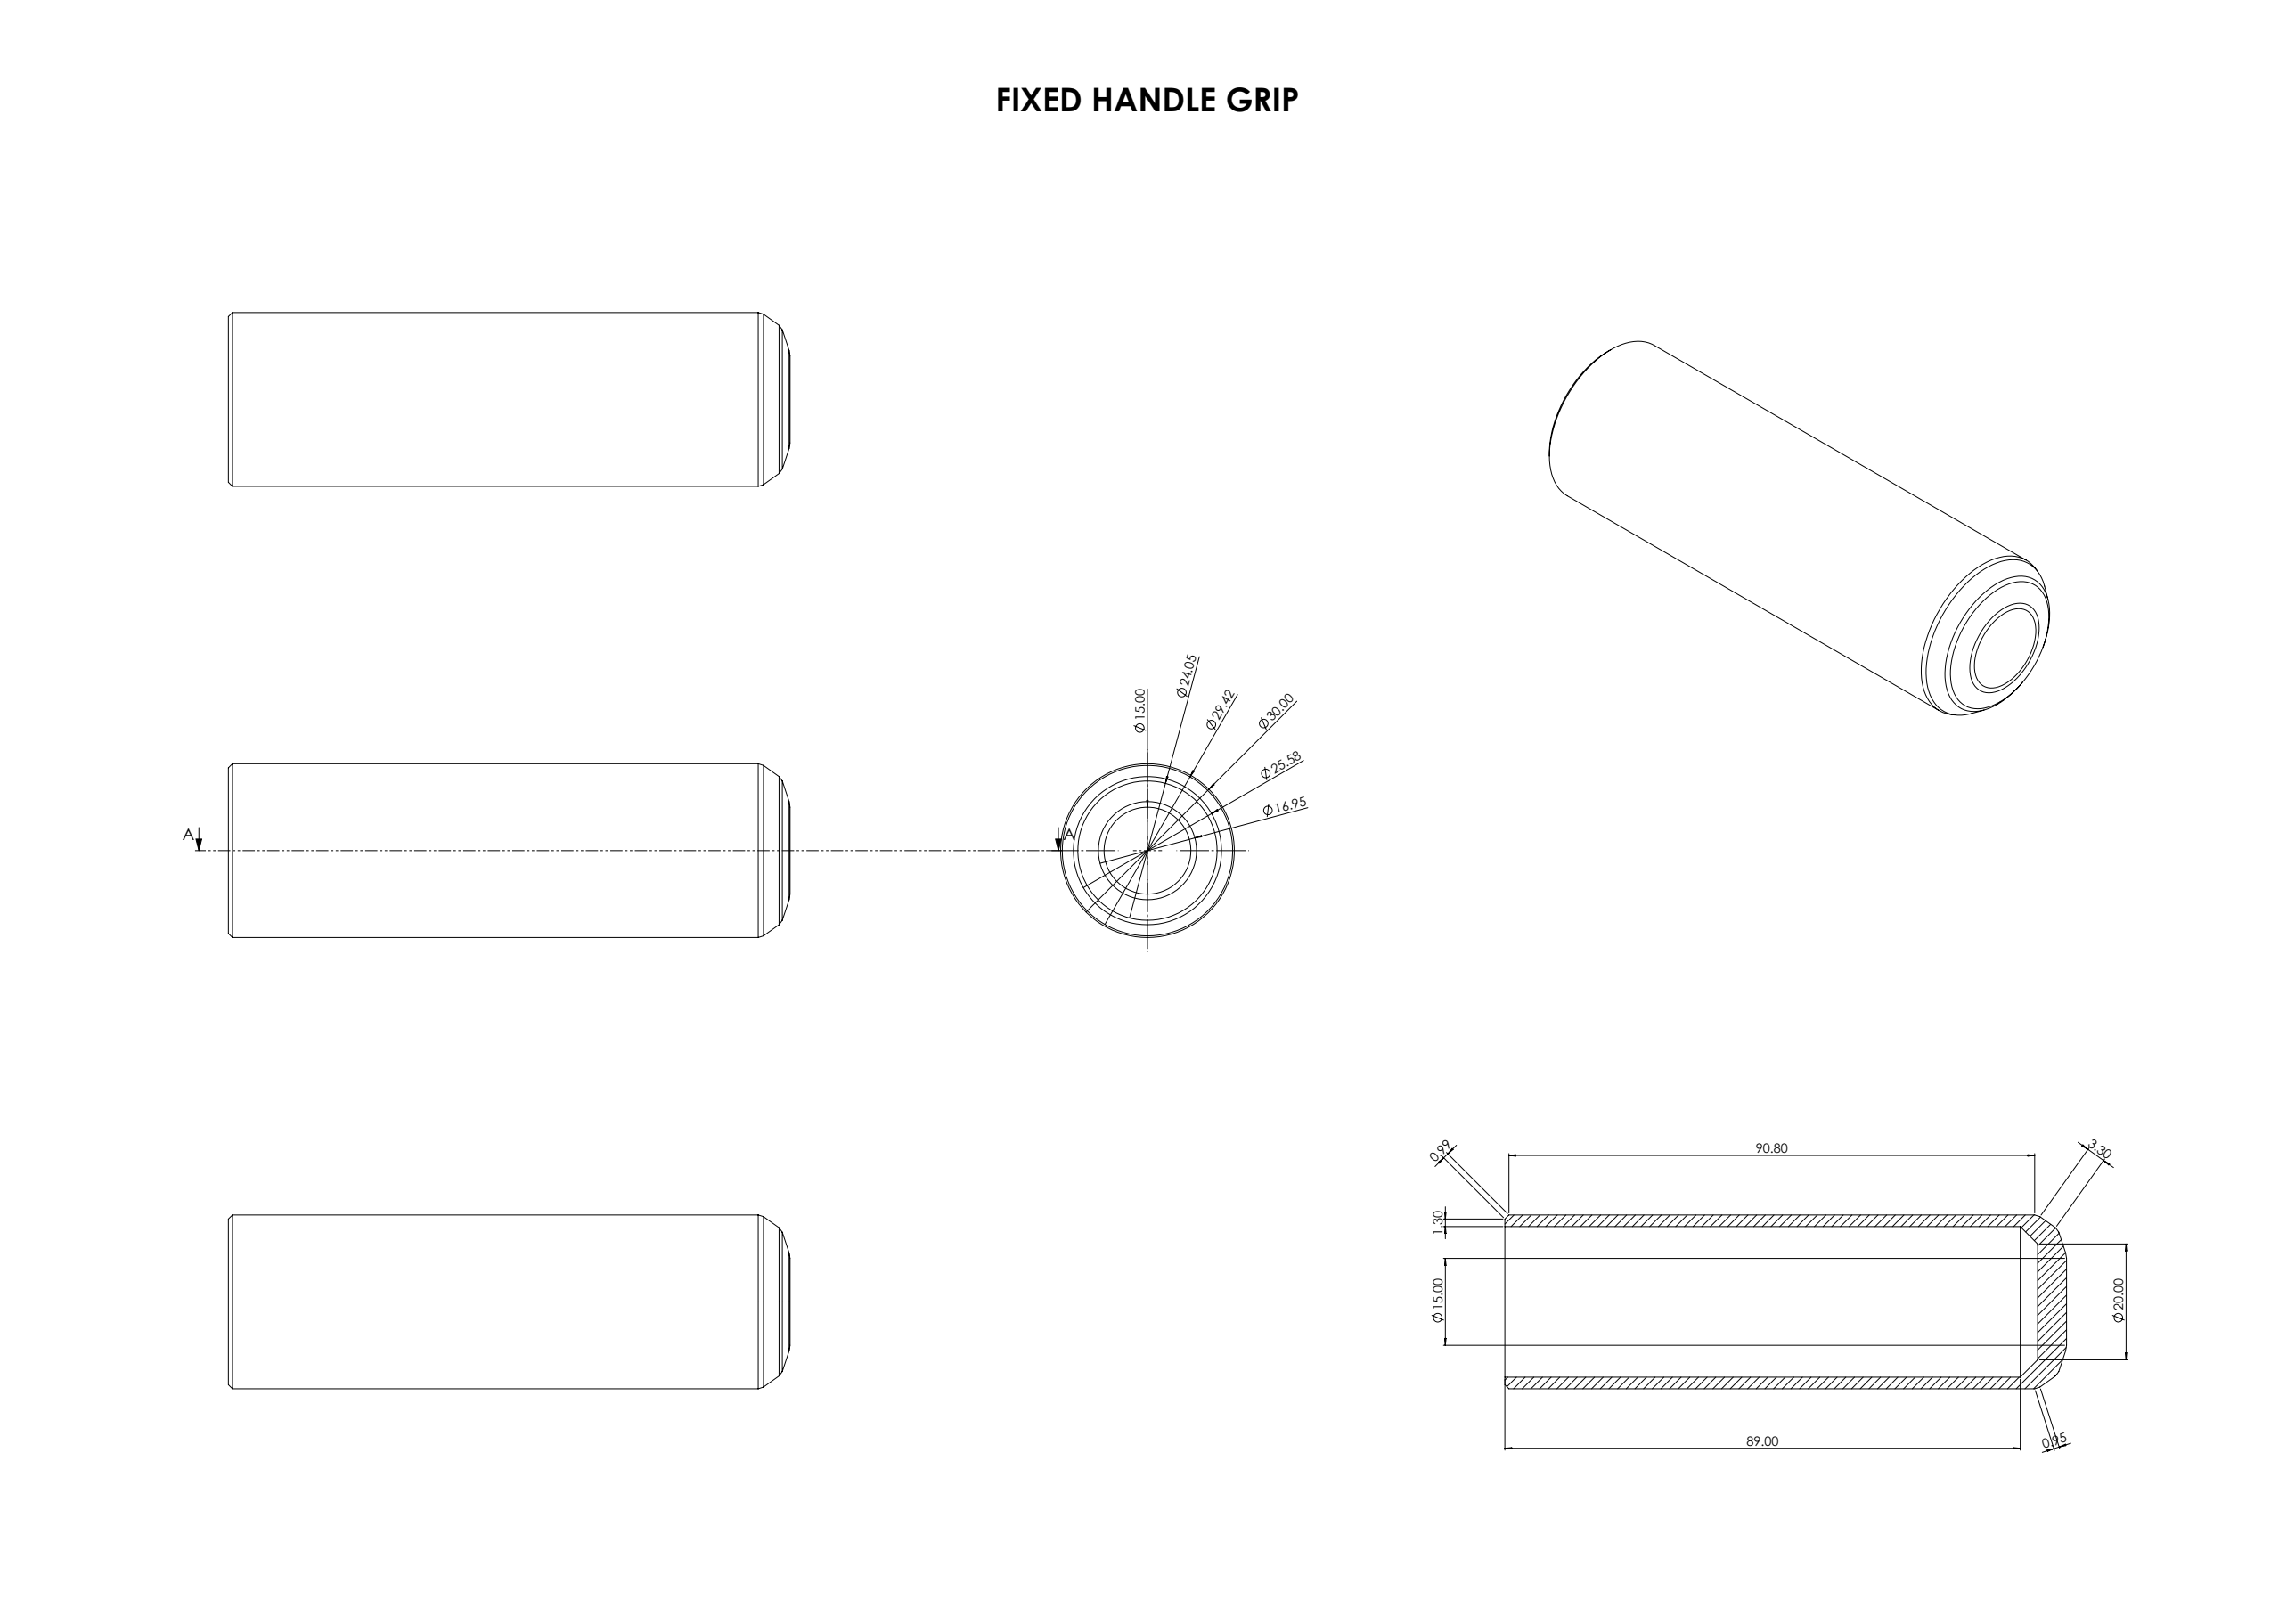
ISO-10303-21;
HEADER;
/* Generated by software containing ST-Developer
 * from STEP Tools, Inc. (www.steptools.com) 
 */

FILE_DESCRIPTION(
/* description */ (''),
/* implementation_level */ '2;1');

FILE_NAME(
/* name */ '19_Fixed_Handle_Grip.step',
/* time_stamp */ '2026-10-26T03:55:20-07:00',
/* author */ (''),
/* organization */ (''),
/* preprocessor_version */ 'ST-DEVELOPER v20.2',
/* originating_system */ 'Autodesk Translation Framework v15.15.0.0',
/* authorisation */ '');

FILE_SCHEMA (('AUTOMOTIVE_DESIGN { 1 0 10303 214 3 1 1 }'));
ENDSEC;

DATA;
#10=MECHANICAL_DESIGN_GEOMETRIC_PRESENTATION_REPRESENTATION('',(#187),#45236);
#147=SHAPE_REPRESENTATION_RELATIONSHIP('SRR','None',#45326,#167);
#167=ADVANCED_BREP_SHAPE_REPRESENTATION('',(#207),#45228);
#187=STYLED_ITEM('',(#45491),#207);
#207=MANIFOLD_SOLID_BREP('Body1',#16529);
#1003=FACE_BOUND('',#3474,.T.);
#1333=PLANE('',#17580);
#1334=PLANE('',#17595);
#1335=PLANE('',#17598);
#1750=CYLINDRICAL_SURFACE('',#17590,15.);
#1751=CYLINDRICAL_SURFACE('',#17592,13.);
#2427=FACE_OUTER_BOUND('',#3465,.T.);
#2428=FACE_OUTER_BOUND('',#3466,.T.);
#2429=FACE_OUTER_BOUND('',#3467,.T.);
#2430=FACE_OUTER_BOUND('',#3468,.T.);
#2431=FACE_OUTER_BOUND('',#3469,.T.);
#2432=FACE_OUTER_BOUND('',#3470,.T.);
#2433=FACE_OUTER_BOUND('',#3471,.T.);
#2434=FACE_OUTER_BOUND('',#3472,.T.);
#2435=FACE_OUTER_BOUND('',#3473,.T.);
#2436=FACE_OUTER_BOUND('',#3475,.T.);
#2437=FACE_OUTER_BOUND('',#3476,.T.);
#2438=FACE_OUTER_BOUND('',#3477,.T.);
#3465=EDGE_LOOP('',(#13800,#13801,#13802,#13803,#13804));
#3466=EDGE_LOOP('',(#13805,#13806,#13807,#13808,#13809,#13810));
#3467=EDGE_LOOP('',(#13811));
#3468=EDGE_LOOP('',(#13812,#13813,#13814,#13815,#13816,#13817));
#3469=EDGE_LOOP('',(#13818,#13819,#13820,#13821,#13822,#13823));
#3470=EDGE_LOOP('',(#13824,#13825,#13826,#13827,#13828,#13829));
#3471=EDGE_LOOP('',(#13830,#13831,#13832,#13833,#13834));
#3472=EDGE_LOOP('',(#13835,#13836,#13837,#13838));
#3473=EDGE_LOOP('',(#13839));
#3474=EDGE_LOOP('',(#13840));
#3475=EDGE_LOOP('',(#13841,#13842,#13843,#13844));
#3476=EDGE_LOOP('',(#13845));
#3477=EDGE_LOOP('',(#13846,#13847,#13848,#13849));
#4667=LINE('',#40590,#5978);
#4668=LINE('',#40596,#5979);
#4669=LINE('',#40603,#5980);
#4670=LINE('',#40609,#5981);
#4671=LINE('',#40615,#5982);
#4672=LINE('',#40621,#5983);
#4673=LINE('',#40627,#5984);
#4674=LINE('',#40633,#5985);
#4675=LINE('',#40638,#5986);
#5978=VECTOR('',#20538,7.98717082451265);
#5979=VECTOR('',#20545,10.25);
#5980=VECTOR('',#20554,12.4081387239171);
#5981=VECTOR('',#20561,13.75);
#5982=VECTOR('',#20568,14.8546904515702);
#5983=VECTOR('',#20575,15.);
#5984=VECTOR('',#20582,13.);
#5985=VECTOR('',#20591,14.65);
#5986=VECTOR('',#20598,11.5);
#6784=CIRCLE('',#17574,7.50000000000002);
#6785=CIRCLE('',#17575,8.47434164902529);
#6786=CIRCLE('',#17576,8.47434164902529);
#6787=CIRCLE('',#17578,12.0256583509747);
#6788=CIRCLE('',#17579,12.0256583509747);
#6789=CIRCLE('',#17582,12.7906190968596);
#6790=CIRCLE('',#17583,12.7906190968596);
#6791=CIRCLE('',#17585,14.7093809031404);
#6792=CIRCLE('',#17586,14.7093809031404);
#6793=CIRCLE('',#17588,15.);
#6794=CIRCLE('',#17589,15.);
#6795=CIRCLE('',#17591,15.);
#6796=CIRCLE('',#17593,13.);
#6797=CIRCLE('',#17594,13.);
#6798=CIRCLE('',#17596,14.3);
#6799=CIRCLE('',#17599,10.);
#7926=VERTEX_POINT('',#40587);
#7927=VERTEX_POINT('',#40589);
#7928=VERTEX_POINT('',#40591);
#7929=VERTEX_POINT('',#40595);
#7930=VERTEX_POINT('',#40597);
#7931=VERTEX_POINT('',#40602);
#7932=VERTEX_POINT('',#40604);
#7933=VERTEX_POINT('',#40608);
#7934=VERTEX_POINT('',#40610);
#7935=VERTEX_POINT('',#40614);
#7936=VERTEX_POINT('',#40616);
#7937=VERTEX_POINT('',#40620);
#7938=VERTEX_POINT('',#40624);
#7939=VERTEX_POINT('',#40626);
#7940=VERTEX_POINT('',#40630);
#7941=VERTEX_POINT('',#40635);
#9963=EDGE_CURVE('',#7926,#7926,#6784,.T.);
#9964=EDGE_CURVE('',#7926,#7927,#4667,.T.);
#9965=EDGE_CURVE('',#7927,#7928,#6785,.T.);
#9966=EDGE_CURVE('',#7928,#7927,#6786,.T.);
#9967=EDGE_CURVE('',#7928,#7929,#4668,.T.);
#9968=EDGE_CURVE('',#7930,#7929,#6787,.T.);
#9969=EDGE_CURVE('',#7929,#7930,#6788,.T.);
#9970=EDGE_CURVE('',#7930,#7931,#4669,.T.);
#9971=EDGE_CURVE('',#7931,#7932,#6789,.T.);
#9972=EDGE_CURVE('',#7932,#7931,#6790,.T.);
#9973=EDGE_CURVE('',#7932,#7933,#4670,.T.);
#9974=EDGE_CURVE('',#7934,#7933,#6791,.T.);
#9975=EDGE_CURVE('',#7933,#7934,#6792,.T.);
#9976=EDGE_CURVE('',#7934,#7935,#4671,.T.);
#9977=EDGE_CURVE('',#7935,#7936,#6793,.T.);
#9978=EDGE_CURVE('',#7936,#7935,#6794,.T.);
#9979=EDGE_CURVE('',#7936,#7937,#4672,.T.);
#9980=EDGE_CURVE('',#7937,#7937,#6795,.T.);
#9981=EDGE_CURVE('',#7938,#7938,#6796,.T.);
#9982=EDGE_CURVE('',#7938,#7939,#4673,.T.);
#9983=EDGE_CURVE('',#7939,#7939,#6797,.T.);
#9984=EDGE_CURVE('',#7940,#7940,#6798,.T.);
#9985=EDGE_CURVE('',#7937,#7940,#4674,.T.);
#9986=EDGE_CURVE('',#7941,#7941,#6799,.T.);
#9987=EDGE_CURVE('',#7941,#7938,#4675,.T.);
#13800=ORIENTED_EDGE('',*,*,#9963,.T.);
#13801=ORIENTED_EDGE('',*,*,#9964,.T.);
#13802=ORIENTED_EDGE('',*,*,#9965,.T.);
#13803=ORIENTED_EDGE('',*,*,#9966,.T.);
#13804=ORIENTED_EDGE('',*,*,#9964,.F.);
#13805=ORIENTED_EDGE('',*,*,#9965,.F.);
#13806=ORIENTED_EDGE('',*,*,#9966,.F.);
#13807=ORIENTED_EDGE('',*,*,#9967,.T.);
#13808=ORIENTED_EDGE('',*,*,#9968,.F.);
#13809=ORIENTED_EDGE('',*,*,#9969,.F.);
#13810=ORIENTED_EDGE('',*,*,#9967,.F.);
#13811=ORIENTED_EDGE('',*,*,#9963,.F.);
#13812=ORIENTED_EDGE('',*,*,#9968,.T.);
#13813=ORIENTED_EDGE('',*,*,#9969,.T.);
#13814=ORIENTED_EDGE('',*,*,#9970,.T.);
#13815=ORIENTED_EDGE('',*,*,#9971,.T.);
#13816=ORIENTED_EDGE('',*,*,#9972,.T.);
#13817=ORIENTED_EDGE('',*,*,#9970,.F.);
#13818=ORIENTED_EDGE('',*,*,#9971,.F.);
#13819=ORIENTED_EDGE('',*,*,#9972,.F.);
#13820=ORIENTED_EDGE('',*,*,#9973,.T.);
#13821=ORIENTED_EDGE('',*,*,#9974,.F.);
#13822=ORIENTED_EDGE('',*,*,#9975,.F.);
#13823=ORIENTED_EDGE('',*,*,#9973,.F.);
#13824=ORIENTED_EDGE('',*,*,#9974,.T.);
#13825=ORIENTED_EDGE('',*,*,#9975,.T.);
#13826=ORIENTED_EDGE('',*,*,#9976,.T.);
#13827=ORIENTED_EDGE('',*,*,#9977,.T.);
#13828=ORIENTED_EDGE('',*,*,#9978,.T.);
#13829=ORIENTED_EDGE('',*,*,#9976,.F.);
#13830=ORIENTED_EDGE('',*,*,#9977,.F.);
#13831=ORIENTED_EDGE('',*,*,#9978,.F.);
#13832=ORIENTED_EDGE('',*,*,#9979,.T.);
#13833=ORIENTED_EDGE('',*,*,#9980,.T.);
#13834=ORIENTED_EDGE('',*,*,#9979,.F.);
#13835=ORIENTED_EDGE('',*,*,#9981,.T.);
#13836=ORIENTED_EDGE('',*,*,#9982,.T.);
#13837=ORIENTED_EDGE('',*,*,#9983,.F.);
#13838=ORIENTED_EDGE('',*,*,#9982,.F.);
#13839=ORIENTED_EDGE('',*,*,#9984,.F.);
#13840=ORIENTED_EDGE('',*,*,#9983,.T.);
#13841=ORIENTED_EDGE('',*,*,#9980,.F.);
#13842=ORIENTED_EDGE('',*,*,#9985,.T.);
#13843=ORIENTED_EDGE('',*,*,#9984,.T.);
#13844=ORIENTED_EDGE('',*,*,#9985,.F.);
#13845=ORIENTED_EDGE('',*,*,#9986,.F.);
#13846=ORIENTED_EDGE('',*,*,#9986,.T.);
#13847=ORIENTED_EDGE('',*,*,#9987,.T.);
#13848=ORIENTED_EDGE('',*,*,#9981,.F.);
#13849=ORIENTED_EDGE('',*,*,#9987,.F.);
#15514=CONICAL_SURFACE('',#17573,7.98717082451265,1.40992104959656);
#15515=CONICAL_SURFACE('',#17577,10.25,1.24904577239826);
#15516=CONICAL_SURFACE('',#17581,12.4081387239171,0.934647629190528);
#15517=CONICAL_SURFACE('',#17584,13.75,0.620249485982819);
#15518=CONICAL_SURFACE('',#17587,14.8546904515702,0.310124742991409);
#15519=CONICAL_SURFACE('',#17597,14.65,0.78539816339747);
#15520=CONICAL_SURFACE('',#17600,11.5,0.785398163397447);
#16155=ADVANCED_FACE('',(#2427),#15514,.T.);
#16156=ADVANCED_FACE('',(#2428),#15515,.T.);
#16157=ADVANCED_FACE('',(#2429),#1333,.T.);
#16158=ADVANCED_FACE('',(#2430),#15516,.T.);
#16159=ADVANCED_FACE('',(#2431),#15517,.T.);
#16160=ADVANCED_FACE('',(#2432),#15518,.T.);
#16161=ADVANCED_FACE('',(#2433),#1750,.T.);
#16162=ADVANCED_FACE('',(#2434),#1751,.F.);
#16163=ADVANCED_FACE('',(#2435,#1003),#1334,.T.);
#16164=ADVANCED_FACE('',(#2436),#15519,.T.);
#16165=ADVANCED_FACE('',(#2437),#1335,.T.);
#16166=ADVANCED_FACE('',(#2438),#15520,.F.);
#16529=CLOSED_SHELL('',(#16155,#16156,#16157,#16158,#16159,#16160,#16161,
#16162,#16163,#16164,#16165,#16166));
#17572=AXIS2_PLACEMENT_3D('',#40585,#20532,#20533);
#17573=AXIS2_PLACEMENT_3D('',#40586,#20534,#20535);
#17574=AXIS2_PLACEMENT_3D('',#40588,#20536,#20537);
#17575=AXIS2_PLACEMENT_3D('',#40592,#20539,#20540);
#17576=AXIS2_PLACEMENT_3D('',#40593,#20541,#20542);
#17577=AXIS2_PLACEMENT_3D('',#40594,#20543,#20544);
#17578=AXIS2_PLACEMENT_3D('',#40598,#20546,#20547);
#17579=AXIS2_PLACEMENT_3D('',#40599,#20548,#20549);
#17580=AXIS2_PLACEMENT_3D('',#40600,#20550,#20551);
#17581=AXIS2_PLACEMENT_3D('',#40601,#20552,#20553);
#17582=AXIS2_PLACEMENT_3D('',#40605,#20555,#20556);
#17583=AXIS2_PLACEMENT_3D('',#40606,#20557,#20558);
#17584=AXIS2_PLACEMENT_3D('',#40607,#20559,#20560);
#17585=AXIS2_PLACEMENT_3D('',#40611,#20562,#20563);
#17586=AXIS2_PLACEMENT_3D('',#40612,#20564,#20565);
#17587=AXIS2_PLACEMENT_3D('',#40613,#20566,#20567);
#17588=AXIS2_PLACEMENT_3D('',#40617,#20569,#20570);
#17589=AXIS2_PLACEMENT_3D('',#40618,#20571,#20572);
#17590=AXIS2_PLACEMENT_3D('',#40619,#20573,#20574);
#17591=AXIS2_PLACEMENT_3D('',#40622,#20576,#20577);
#17592=AXIS2_PLACEMENT_3D('',#40623,#20578,#20579);
#17593=AXIS2_PLACEMENT_3D('',#40625,#20580,#20581);
#17594=AXIS2_PLACEMENT_3D('',#40628,#20583,#20584);
#17595=AXIS2_PLACEMENT_3D('',#40629,#20585,#20586);
#17596=AXIS2_PLACEMENT_3D('',#40631,#20587,#20588);
#17597=AXIS2_PLACEMENT_3D('',#40632,#20589,#20590);
#17598=AXIS2_PLACEMENT_3D('',#40634,#20592,#20593);
#17599=AXIS2_PLACEMENT_3D('',#40636,#20594,#20595);
#17600=AXIS2_PLACEMENT_3D('',#40637,#20596,#20597);
#20532=DIRECTION('axis',(0.,0.,1.));
#20533=DIRECTION('refdir',(1.,0.,0.));
#20534=DIRECTION('center_axis',(-1.,0.,-3.28183559150414E-15));
#20535=DIRECTION('ref_axis',(0.,-1.,-3.24835777379068E-17));
#20536=DIRECTION('center_axis',(-1.,0.,0.));
#20537=DIRECTION('ref_axis',(0.,-1.,0.));
#20538=DIRECTION('',(-0.16018224300698,0.987087457637495,-3.72744304515565E-16));
#20539=DIRECTION('center_axis',(1.,0.,0.));
#20540=DIRECTION('ref_axis',(0.,-1.,-6.12323399573677E-17));
#20541=DIRECTION('center_axis',(1.,0.,0.));
#20542=DIRECTION('ref_axis',(0.,-1.,-6.12323399573677E-17));
#20543=DIRECTION('center_axis',(-1.,0.,0.));
#20544=DIRECTION('ref_axis',(0.,1.,0.));
#20545=DIRECTION('',(-0.316227766016835,-0.948683298050515,-1.16180196436212E-16));
#20546=DIRECTION('center_axis',(-1.,0.,0.));
#20547=DIRECTION('ref_axis',(0.,-1.,-6.12323399573676E-17));
#20548=DIRECTION('center_axis',(-1.,0.,0.));
#20549=DIRECTION('ref_axis',(0.,-1.,-6.12323399573676E-17));
#20550=DIRECTION('center_axis',(1.,0.,0.));
#20551=DIRECTION('ref_axis',(0.,0.,-1.));
#20552=DIRECTION('center_axis',(-1.,0.,-8.29060943031117E-17));
#20553=DIRECTION('ref_axis',(0.,-1.,-6.12323399573677E-17));
#20554=DIRECTION('',(-0.594101906730864,0.804389783885121,9.85093374101743E-17));
#20555=DIRECTION('center_axis',(1.,0.,0.));
#20556=DIRECTION('ref_axis',(0.,-1.,-6.12323399573677E-17));
#20557=DIRECTION('center_axis',(1.,0.,0.));
#20558=DIRECTION('ref_axis',(0.,-1.,-6.12323399573677E-17));
#20559=DIRECTION('center_axis',(-1.,0.,0.));
#20560=DIRECTION('ref_axis',(0.,1.,0.));
#20561=DIRECTION('',(-0.813733471206736,-0.581238193719095,-7.11811493480279E-17));
#20562=DIRECTION('center_axis',(-1.,0.,0.));
#20563=DIRECTION('ref_axis',(0.,-1.,-6.12323399573677E-17));
#20564=DIRECTION('center_axis',(-1.,0.,0.));
#20565=DIRECTION('ref_axis',(0.,-1.,-6.12323399573677E-17));
#20566=DIRECTION('center_axis',(-1.,0.,9.93188719646043E-16));
#20567=DIRECTION('ref_axis',(0.,-1.,-3.03166806120925E-17));
#20568=DIRECTION('',(-0.952295508549404,0.305177431007982,9.92434579972342E-16));
#20569=DIRECTION('center_axis',(1.,0.,0.));
#20570=DIRECTION('ref_axis',(0.,-1.,0.));
#20571=DIRECTION('center_axis',(1.,0.,0.));
#20572=DIRECTION('ref_axis',(0.,-1.,0.));
#20573=DIRECTION('center_axis',(1.,0.,0.));
#20574=DIRECTION('ref_axis',(0.,1.,0.));
#20575=DIRECTION('',(-1.,0.,0.));
#20576=DIRECTION('center_axis',(1.,0.,0.));
#20577=DIRECTION('ref_axis',(0.,0.,-1.));
#20578=DIRECTION('center_axis',(1.,0.,0.));
#20579=DIRECTION('ref_axis',(0.,1.,0.));
#20580=DIRECTION('center_axis',(1.,0.,0.));
#20581=DIRECTION('ref_axis',(0.,0.,-1.));
#20582=DIRECTION('',(-1.,0.,0.));
#20583=DIRECTION('center_axis',(1.,0.,0.));
#20584=DIRECTION('ref_axis',(0.,0.,-1.));
#20585=DIRECTION('center_axis',(-1.,0.,0.));
#20586=DIRECTION('ref_axis',(0.,0.,1.));
#20587=DIRECTION('center_axis',(1.,0.,0.));
#20588=DIRECTION('ref_axis',(0.,0.,-1.));
#20589=DIRECTION('center_axis',(1.,0.,0.));
#20590=DIRECTION('ref_axis',(0.,1.,0.));
#20591=DIRECTION('',(-0.707106781186532,0.707106781186563,8.65956056235512E-17));
#20592=DIRECTION('center_axis',(-1.,0.,0.));
#20593=DIRECTION('ref_axis',(0.,0.,1.));
#20594=DIRECTION('center_axis',(1.,0.,0.));
#20595=DIRECTION('ref_axis',(0.,0.,-1.));
#20596=DIRECTION('center_axis',(-1.,0.,0.));
#20597=DIRECTION('ref_axis',(0.,1.,0.));
#20598=DIRECTION('',(-0.707106781186548,-0.707106781186547,-8.65956056235492E-17));
#40585=CARTESIAN_POINT('',(0.,0.,0.));
#40586=CARTESIAN_POINT('Origin',(304.920943058496,0.,-2.59451884383998E-16));
#40587=CARTESIAN_POINT('',(305.,7.50000000000002,-9.18485099360518E-16));
#40588=CARTESIAN_POINT('Origin',(305.,0.,0.));
#40589=CARTESIAN_POINT('',(304.841886116992,8.47434164902529,1.03780753753599E-15));
#40590=CARTESIAN_POINT('',(304.920943058496,7.98717082451265,9.78146318448255E-16));
#40591=CARTESIAN_POINT('',(304.841886116992,-8.47434164902529,-1.03780753753599E-15));
#40592=CARTESIAN_POINT('Origin',(304.841886116992,0.,-5.18903768767996E-16));
#40593=CARTESIAN_POINT('Origin',(304.841886116992,0.,-5.18903768767996E-16));
#40594=CARTESIAN_POINT('Origin',(304.25,0.,0.));
#40595=CARTESIAN_POINT('',(303.658113883008,-12.0256583509747,-1.47271840071608E-15));
#40596=CARTESIAN_POINT('',(304.25,-10.25,-1.25526296912604E-15));
#40597=CARTESIAN_POINT('',(303.658113883008,12.0256583509747,-1.47271840071608E-15));
#40598=CARTESIAN_POINT('Origin',(303.658113883008,0.,-7.36359200358042E-16));
#40599=CARTESIAN_POINT('Origin',(303.658113883008,0.,-7.36359200358042E-16));
#40600=CARTESIAN_POINT('Origin',(305.,0.,0.));
#40601=CARTESIAN_POINT('Origin',(303.375623573703,0.,-7.59779368581073E-16));
#40602=CARTESIAN_POINT('',(303.093133264397,12.7906190968596,1.56639907360821E-15));
#40603=CARTESIAN_POINT('',(303.375623573703,12.4081387239171,1.51955873716215E-15));
#40604=CARTESIAN_POINT('',(303.093133264397,-12.7906190968596,-1.56639907360821E-15));
#40605=CARTESIAN_POINT('Origin',(303.093133264397,0.,-7.83199536804103E-16));
#40606=CARTESIAN_POINT('Origin',(303.093133264397,0.,-7.83199536804103E-16));
#40607=CARTESIAN_POINT('Origin',(301.75,0.,0.));
#40608=CARTESIAN_POINT('',(300.406866735603,-14.7093809031404,-1.80137962404702E-15));
#40609=CARTESIAN_POINT('',(301.75,-13.75,-1.68388934882761E-15));
#40610=CARTESIAN_POINT('',(300.406866735603,14.7093809031404,-1.80137962404702E-15));
#40611=CARTESIAN_POINT('Origin',(300.406866735603,0.,-9.00689812023508E-16));
#40612=CARTESIAN_POINT('Origin',(300.406866735603,0.,-9.00689812023508E-16));
#40613=CARTESIAN_POINT('Origin',(299.953433367802,0.,-4.50344906011754E-16));
#40614=CARTESIAN_POINT('',(299.5,15.,1.83697019872103E-15));
#40615=CARTESIAN_POINT('',(299.953433367802,14.8546904515702,1.81917491138402E-15));
#40616=CARTESIAN_POINT('',(299.5,-15.,-1.83697019872103E-15));
#40617=CARTESIAN_POINT('Origin',(299.5,0.,0.));
#40618=CARTESIAN_POINT('Origin',(299.5,0.,0.));
#40619=CARTESIAN_POINT('Origin',(254.35,0.,0.));
#40620=CARTESIAN_POINT('',(208.7,-15.,-1.83697019872103E-15));
#40621=CARTESIAN_POINT('',(254.35,-15.,-1.83697019872103E-15));
#40622=CARTESIAN_POINT('Origin',(208.7,0.,0.));
#40623=CARTESIAN_POINT('Origin',(252.5,0.,0.));
#40624=CARTESIAN_POINT('',(297.,-13.,-1.59204083889156E-15));
#40625=CARTESIAN_POINT('Origin',(297.,0.,0.));
#40626=CARTESIAN_POINT('',(208.,-13.,-1.59204083889156E-15));
#40627=CARTESIAN_POINT('',(252.5,-13.,-1.59204083889156E-15));
#40628=CARTESIAN_POINT('Origin',(208.,0.,0.));
#40629=CARTESIAN_POINT('Origin',(208.,14.3,0.));
#40630=CARTESIAN_POINT('',(208.,-14.3,-1.75124492278071E-15));
#40631=CARTESIAN_POINT('Origin',(208.,0.,0.));
#40632=CARTESIAN_POINT('Origin',(208.35,0.,0.));
#40633=CARTESIAN_POINT('',(208.35,-14.65,-1.79410756075087E-15));
#40634=CARTESIAN_POINT('Origin',(300.,10.,0.));
#40635=CARTESIAN_POINT('',(300.,-10.,-1.22464679914735E-15));
#40636=CARTESIAN_POINT('Origin',(300.,0.,0.));
#40637=CARTESIAN_POINT('Origin',(298.5,0.,0.));
#40638=CARTESIAN_POINT('',(298.5,-11.5,-1.40834381901946E-15));
#45206=UNCERTAINTY_MEASURE_WITH_UNIT(LENGTH_MEASURE(0.01),#45237,
'DISTANCE_ACCURACY_VALUE',
'Maximum model space distance between geometric entities at asserted c
onnectivities');
#45214=UNCERTAINTY_MEASURE_WITH_UNIT(LENGTH_MEASURE(0.01),#45237,
'DISTANCE_ACCURACY_VALUE',
'Maximum model space distance between geometric entities at asserted c
onnectivities');
#45228=(
GEOMETRIC_REPRESENTATION_CONTEXT(3)
GLOBAL_UNCERTAINTY_ASSIGNED_CONTEXT((#45206))
GLOBAL_UNIT_ASSIGNED_CONTEXT((#45237,#45239,#45240))
REPRESENTATION_CONTEXT('','3D')
);
#45236=(
GEOMETRIC_REPRESENTATION_CONTEXT(3)
GLOBAL_UNCERTAINTY_ASSIGNED_CONTEXT((#45214))
GLOBAL_UNIT_ASSIGNED_CONTEXT((#45237,#45239,#45240))
REPRESENTATION_CONTEXT('','3D')
);
#45237=(
LENGTH_UNIT()
NAMED_UNIT(*)
SI_UNIT(.MILLI.,.METRE.)
);
#45239=(
NAMED_UNIT(*)
PLANE_ANGLE_UNIT()
SI_UNIT($,.RADIAN.)
);
#45240=(
NAMED_UNIT(*)
SI_UNIT($,.STERADIAN.)
SOLID_ANGLE_UNIT()
);
#45254=SHAPE_DEFINITION_REPRESENTATION(#45275,#45326);
#45275=PRODUCT_DEFINITION_SHAPE('',$,#45348);
#45326=SHAPE_REPRESENTATION('',(#17572),#45228);
#45334=PRODUCT_DEFINITION_CONTEXT('part definition',#45399,'design');
#45348=PRODUCT_DEFINITION('2026-10-25-23-38-29-621',
'19_Fixed_Handle_Grip',#45369,#45334);
#45369=PRODUCT_DEFINITION_FORMATION('',$,#45414);
#45399=APPLICATION_CONTEXT(
'Core Data for Automotive Mechanical Design Process');
#45400=PRODUCT_CONTEXT('part definition',#45399,'mechanical');
#45414=PRODUCT('2026-10-25-23-38-29-621','19_Fixed_Handle_Grip',$,(#45400));
#45485=COLOUR_RGB('Black',0.12,0.14,0.17);
#45486=FILL_AREA_STYLE_COLOUR('',#45485);
#45487=FILL_AREA_STYLE('',(#45486));
#45488=SURFACE_STYLE_FILL_AREA(#45487);
#45489=SURFACE_SIDE_STYLE('',(#45488));
#45490=SURFACE_STYLE_USAGE(.BOTH.,#45489);
#45491=PRESENTATION_STYLE_ASSIGNMENT((#45490));
ENDSEC;
END-ISO-10303-21;
